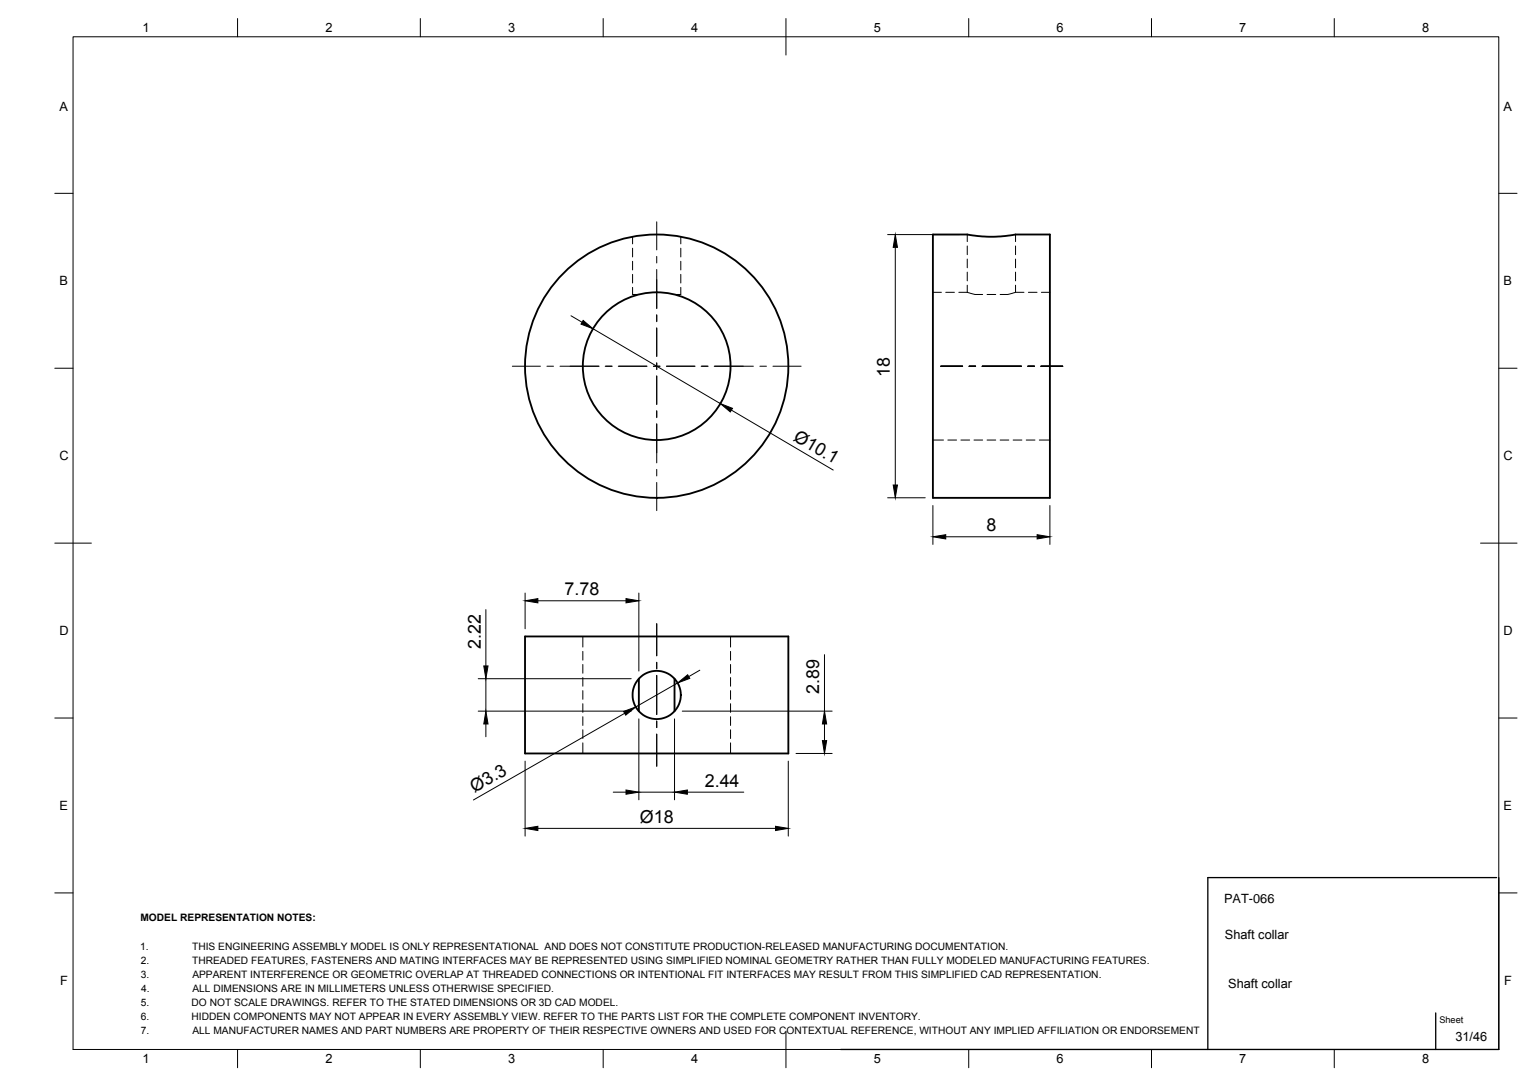
ISO-10303-21;
HEADER;
/* Generated by software containing ST-Developer
 * from STEP Tools, Inc. (www.steptools.com) 
 */

FILE_DESCRIPTION(
/* description */ ('Lever-operated bar clamp (toggle)'),
/* implementation_level */ '2;1');

FILE_NAME(
/* name */ 'Shaft collar.step',
/* time_stamp */ '2026-10-28T03:25:02-07:00',
/* author */ (''),
/* organization */ (''),
/* preprocessor_version */ 'ST-DEVELOPER v20.2',
/* originating_system */ 'Autodesk Translation Framework v15.17.0.0',
/* authorisation */ '');

FILE_SCHEMA (('AUTOMOTIVE_DESIGN { 1 0 10303 214 3 1 1 }'));
ENDSEC;

DATA;
#10=MECHANICAL_DESIGN_GEOMETRIC_PRESENTATION_REPRESENTATION('',(#440),#12413);
#281=B_SPLINE_CURVE_WITH_KNOTS('',3,(#11610,#11611,#11612,#11613,#11614,
#11615,#11616,#11617,#11618,#11619,#11620,#11621,#11622,#11623),
 .UNSPECIFIED.,.F.,.F.,(4,2,2,2,2,2,4),(0.618551524396288,0.626563103102763,
0.689203386094986,0.751843669087208,0.814483952079431,0.877124235071654,
0.88513581377813),.UNSPECIFIED.);
#282=B_SPLINE_CURVE_WITH_KNOTS('',3,(#11629,#11630,#11631,#11632,#11633,
#11634,#11635,#11636,#11637,#11638,#11639,#11640,#11641,#11642,#11643,#11644,
#11645,#11646),.UNSPECIFIED.,.F.,.F.,(4,2,2,2,2,2,2,2,4),(0.,0.0623062782223138,
0.124612556444628,0.186916384615148,0.249220212785668,0.311524040956189,
0.373827869126709,0.436134147349023,0.498440425571337),.UNSPECIFIED.);
#283=B_SPLINE_CURVE_WITH_KNOTS('',3,(#11647,#11648,#11649,#11650,#11651,
#11652,#11653,#11654,#11655,#11656,#11657,#11658,#11659,#11660,#11661,#11662,
#11663,#11664),.UNSPECIFIED.,.F.,.F.,(4,2,2,2,2,2,2,2,4),(0.498440425571337,
0.560746703793651,0.623052982015964,0.685356810186485,0.747660638357005,
0.809964466527525,0.872268294698046,0.93457457292036,0.996880851142673),
 .UNSPECIFIED.);
#284=B_SPLINE_CURVE_WITH_KNOTS('',3,(#11667,#11668,#11669,#11670,#11671,
#11672,#11673,#11674,#11675,#11676,#11677,#11678,#11679,#11680),
 .UNSPECIFIED.,.F.,.F.,(4,2,2,2,2,2,4),(0.117322411671483,0.125333990377957,
0.18797427337018,0.250614556362403,0.313254839354626,0.375895122346849,
0.383906701053325),.UNSPECIFIED.);
#356=SHAPE_REPRESENTATION_RELATIONSHIP('SRR','None',#12598,#394);
#394=ADVANCED_BREP_SHAPE_REPRESENTATION('',(#485),#12395);
#440=STYLED_ITEM('',(#12869),#485);
#485=MANIFOLD_SOLID_BREP('Body1',#6601);
#617=FACE_BOUND('',#1683,.T.);
#618=FACE_BOUND('',#1685,.T.);
#619=FACE_BOUND('',#1687,.T.);
#620=FACE_BOUND('',#1689,.T.);
#798=PLANE('',#7591);
#799=PLANE('',#7596);
#800=PLANE('',#7603);
#801=PLANE('',#7604);
#1156=FACE_OUTER_BOUND('',#1679,.T.);
#1157=FACE_OUTER_BOUND('',#1680,.T.);
#1158=FACE_OUTER_BOUND('',#1681,.T.);
#1159=FACE_OUTER_BOUND('',#1682,.T.);
#1160=FACE_OUTER_BOUND('',#1684,.T.);
#1161=FACE_OUTER_BOUND('',#1686,.T.);
#1162=FACE_OUTER_BOUND('',#1688,.T.);
#1679=EDGE_LOOP('',(#5513,#5514));
#1680=EDGE_LOOP('',(#5515,#5516,#5517,#5518,#5519,#5520,#5521,#5522,#5523));
#1681=EDGE_LOOP('',(#5524,#5525,#5526));
#1682=EDGE_LOOP('',(#5527,#5528,#5529,#5530));
#1683=EDGE_LOOP('',(#5531,#5532,#5533,#5534));
#1684=EDGE_LOOP('',(#5535,#5536,#5537,#5538));
#1685=EDGE_LOOP('',(#5539,#5540));
#1686=EDGE_LOOP('',(#5541));
#1687=EDGE_LOOP('',(#5542));
#1688=EDGE_LOOP('',(#5543));
#1689=EDGE_LOOP('',(#5544));
#2130=LINE('',#11606,#2571);
#2131=LINE('',#11627,#2572);
#2132=LINE('',#11682,#2573);
#2133=LINE('',#11687,#2574);
#2134=LINE('',#11693,#2575);
#2571=VECTOR('',#9279,1.);
#2572=VECTOR('',#9286,0.164999999999999);
#2573=VECTOR('',#9291,1.);
#2574=VECTOR('',#9296,0.505);
#2575=VECTOR('',#9303,0.9);
#2982=CIRCLE('',#7592,0.164999999999999);
#2983=CIRCLE('',#7594,0.164999999999999);
#2984=CIRCLE('',#7595,0.164999999999999);
#2985=CIRCLE('',#7598,0.505);
#2986=CIRCLE('',#7599,0.505);
#2987=CIRCLE('',#7601,0.9);
#2988=CIRCLE('',#7602,0.9);
#3445=VERTEX_POINT('',#11604);
#3446=VERTEX_POINT('',#11605);
#3447=VERTEX_POINT('',#11609);
#3448=VERTEX_POINT('',#11624);
#3449=VERTEX_POINT('',#11626);
#3450=VERTEX_POINT('',#11628);
#3451=VERTEX_POINT('',#11665);
#3452=VERTEX_POINT('',#11684);
#3453=VERTEX_POINT('',#11686);
#3454=VERTEX_POINT('',#11690);
#3455=VERTEX_POINT('',#11692);
#4161=EDGE_CURVE('',#3445,#3446,#2130,.T.);
#4162=EDGE_CURVE('',#3445,#3446,#2982,.T.);
#4163=EDGE_CURVE('',#3447,#3445,#281,.T.);
#4164=EDGE_CURVE('',#3448,#3447,#2983,.T.);
#4165=EDGE_CURVE('',#3448,#3449,#2131,.T.);
#4166=EDGE_CURVE('',#3450,#3449,#282,.T.);
#4167=EDGE_CURVE('',#3449,#3450,#283,.T.);
#4168=EDGE_CURVE('',#3451,#3448,#2984,.T.);
#4169=EDGE_CURVE('',#3446,#3451,#284,.T.);
#4170=EDGE_CURVE('',#3451,#3447,#2132,.T.);
#4171=EDGE_CURVE('',#3452,#3452,#2985,.T.);
#4172=EDGE_CURVE('',#3452,#3453,#2133,.T.);
#4173=EDGE_CURVE('',#3453,#3453,#2986,.T.);
#4174=EDGE_CURVE('',#3454,#3454,#2987,.T.);
#4175=EDGE_CURVE('',#3454,#3455,#2134,.T.);
#4176=EDGE_CURVE('',#3455,#3455,#2988,.T.);
#5513=ORIENTED_EDGE('',*,*,#4161,.F.);
#5514=ORIENTED_EDGE('',*,*,#4162,.T.);
#5515=ORIENTED_EDGE('',*,*,#4163,.F.);
#5516=ORIENTED_EDGE('',*,*,#4164,.F.);
#5517=ORIENTED_EDGE('',*,*,#4165,.T.);
#5518=ORIENTED_EDGE('',*,*,#4166,.F.);
#5519=ORIENTED_EDGE('',*,*,#4167,.F.);
#5520=ORIENTED_EDGE('',*,*,#4165,.F.);
#5521=ORIENTED_EDGE('',*,*,#4168,.F.);
#5522=ORIENTED_EDGE('',*,*,#4169,.F.);
#5523=ORIENTED_EDGE('',*,*,#4162,.F.);
#5524=ORIENTED_EDGE('',*,*,#4170,.F.);
#5525=ORIENTED_EDGE('',*,*,#4168,.T.);
#5526=ORIENTED_EDGE('',*,*,#4164,.T.);
#5527=ORIENTED_EDGE('',*,*,#4171,.F.);
#5528=ORIENTED_EDGE('',*,*,#4172,.T.);
#5529=ORIENTED_EDGE('',*,*,#4173,.T.);
#5530=ORIENTED_EDGE('',*,*,#4172,.F.);
#5531=ORIENTED_EDGE('',*,*,#4169,.T.);
#5532=ORIENTED_EDGE('',*,*,#4170,.T.);
#5533=ORIENTED_EDGE('',*,*,#4163,.T.);
#5534=ORIENTED_EDGE('',*,*,#4161,.T.);
#5535=ORIENTED_EDGE('',*,*,#4174,.F.);
#5536=ORIENTED_EDGE('',*,*,#4175,.T.);
#5537=ORIENTED_EDGE('',*,*,#4176,.T.);
#5538=ORIENTED_EDGE('',*,*,#4175,.F.);
#5539=ORIENTED_EDGE('',*,*,#4166,.T.);
#5540=ORIENTED_EDGE('',*,*,#4167,.T.);
#5541=ORIENTED_EDGE('',*,*,#4174,.T.);
#5542=ORIENTED_EDGE('',*,*,#4171,.T.);
#5543=ORIENTED_EDGE('',*,*,#4176,.F.);
#5544=ORIENTED_EDGE('',*,*,#4173,.F.);
#6125=CYLINDRICAL_SURFACE('',#7593,0.164999999999999);
#6126=CYLINDRICAL_SURFACE('',#7597,0.505);
#6127=CYLINDRICAL_SURFACE('',#7600,0.9);
#6431=ADVANCED_FACE('',(#1156),#798,.T.);
#6432=ADVANCED_FACE('',(#1157),#6125,.F.);
#6433=ADVANCED_FACE('',(#1158),#799,.T.);
#6434=ADVANCED_FACE('',(#1159,#617),#6126,.F.);
#6435=ADVANCED_FACE('',(#1160,#618),#6127,.T.);
#6436=ADVANCED_FACE('',(#1161,#619),#800,.T.);
#6437=ADVANCED_FACE('',(#1162,#620),#801,.F.);
#6601=CLOSED_SHELL('',(#6431,#6432,#6433,#6434,#6435,#6436,#6437));
#7590=AXIS2_PLACEMENT_3D('',#11602,#9275,#9276);
#7591=AXIS2_PLACEMENT_3D('',#11603,#9277,#9278);
#7592=AXIS2_PLACEMENT_3D('',#11607,#9280,#9281);
#7593=AXIS2_PLACEMENT_3D('',#11608,#9282,#9283);
#7594=AXIS2_PLACEMENT_3D('',#11625,#9284,#9285);
#7595=AXIS2_PLACEMENT_3D('',#11666,#9287,#9288);
#7596=AXIS2_PLACEMENT_3D('',#11681,#9289,#9290);
#7597=AXIS2_PLACEMENT_3D('',#11683,#9292,#9293);
#7598=AXIS2_PLACEMENT_3D('',#11685,#9294,#9295);
#7599=AXIS2_PLACEMENT_3D('',#11688,#9297,#9298);
#7600=AXIS2_PLACEMENT_3D('',#11689,#9299,#9300);
#7601=AXIS2_PLACEMENT_3D('',#11691,#9301,#9302);
#7602=AXIS2_PLACEMENT_3D('',#11694,#9304,#9305);
#7603=AXIS2_PLACEMENT_3D('',#11695,#9306,#9307);
#7604=AXIS2_PLACEMENT_3D('',#11696,#9308,#9309);
#9275=DIRECTION('axis',(0.,0.,1.));
#9276=DIRECTION('refdir',(1.,0.,0.));
#9277=DIRECTION('center_axis',(1.,0.,0.));
#9278=DIRECTION('ref_axis',(0.,0.,-1.));
#9279=DIRECTION('',(0.,1.,0.));
#9280=DIRECTION('center_axis',(1.,0.,0.));
#9281=DIRECTION('ref_axis',(0.,0.,-1.));
#9282=DIRECTION('center_axis',(1.,0.,0.));
#9283=DIRECTION('ref_axis',(0.,0.,-1.));
#9284=DIRECTION('center_axis',(1.,0.,0.));
#9285=DIRECTION('ref_axis',(0.,0.,-1.));
#9286=DIRECTION('',(1.,0.,0.));
#9287=DIRECTION('center_axis',(1.,0.,0.));
#9288=DIRECTION('ref_axis',(0.,0.,-1.));
#9289=DIRECTION('center_axis',(1.,0.,0.));
#9290=DIRECTION('ref_axis',(0.,0.,-1.));
#9291=DIRECTION('',(0.,-1.,0.));
#9292=DIRECTION('center_axis',(0.,1.,0.));
#9293=DIRECTION('ref_axis',(1.,0.,0.));
#9294=DIRECTION('center_axis',(0.,-1.,0.));
#9295=DIRECTION('ref_axis',(1.,0.,0.));
#9296=DIRECTION('',(0.,-1.,0.));
#9297=DIRECTION('center_axis',(0.,-1.,0.));
#9298=DIRECTION('ref_axis',(1.,0.,0.));
#9299=DIRECTION('center_axis',(0.,1.,0.));
#9300=DIRECTION('ref_axis',(1.,0.,0.));
#9301=DIRECTION('center_axis',(0.,1.,0.));
#9302=DIRECTION('ref_axis',(1.,0.,0.));
#9303=DIRECTION('',(0.,-1.,0.));
#9304=DIRECTION('center_axis',(0.,1.,0.));
#9305=DIRECTION('ref_axis',(1.,0.,0.));
#9306=DIRECTION('center_axis',(0.,1.,0.));
#9307=DIRECTION('ref_axis',(1.,0.,0.));
#9308=DIRECTION('center_axis',(0.,1.,0.));
#9309=DIRECTION('ref_axis',(1.,0.,0.));
#11602=CARTESIAN_POINT('',(0.,0.,0.));
#11603=CARTESIAN_POINT('Origin',(-3.51,1.4,11.));
#11604=CARTESIAN_POINT('',(-3.51,1.28909463493591,10.8778320827713));
#11605=CARTESIAN_POINT('',(-3.51,1.51090536506409,10.8778320827713));
#11606=CARTESIAN_POINT('',(-3.51,1.,10.8778320827713));
#11607=CARTESIAN_POINT('Origin',(-3.51,1.4,11.));
#11608=CARTESIAN_POINT('Origin',(-3.51,1.4,11.));
#11609=CARTESIAN_POINT('',(-3.51,1.28909463493591,11.1221679172287));
#11610=CARTESIAN_POINT('Ctrl Pts',(-3.51,1.28909463493591,11.1221679172287));
#11611=CARTESIAN_POINT('Ctrl Pts',(-3.50955146832001,1.28711294069536,11.1203689136263));
#11612=CARTESIAN_POINT('Ctrl Pts',(-3.50910475462832,1.28518965877367,11.1185348965652));
#11613=CARTESIAN_POINT('Ctrl Pts',(-3.50520498446835,1.2687667552278,11.1021119930194));
#11614=CARTESIAN_POINT('Ctrl Pts',(-3.50155748539241,1.25609154388858,11.0836597150224));
#11615=CARTESIAN_POINT('Ctrl Pts',(-3.49642218023894,1.23920409039234,11.0430495960472));
#11616=CARTESIAN_POINT('Ctrl Pts',(-3.495,1.235,11.0208800943307));
#11617=CARTESIAN_POINT('Ctrl Pts',(-3.495,1.235,10.9791199056693));
#11618=CARTESIAN_POINT('Ctrl Pts',(-3.49642218023894,1.23920409039234,10.9569504039528));
#11619=CARTESIAN_POINT('Ctrl Pts',(-3.50155748539241,1.25609154388858,10.9163402849776));
#11620=CARTESIAN_POINT('Ctrl Pts',(-3.50520498446835,1.2687667552278,10.8978880069806));
#11621=CARTESIAN_POINT('Ctrl Pts',(-3.50910475462832,1.28518965877367,10.8814651034348));
#11622=CARTESIAN_POINT('Ctrl Pts',(-3.50955146832001,1.28711294069536,10.8796310863737));
#11623=CARTESIAN_POINT('Ctrl Pts',(-3.51,1.28909463493591,10.8778320827713));
#11624=CARTESIAN_POINT('',(-3.51,1.4,11.165));
#11625=CARTESIAN_POINT('Origin',(-3.51,1.4,11.));
#11626=CARTESIAN_POINT('',(-3.11525427381648,1.4,11.165));
#11627=CARTESIAN_POINT('',(-3.51,1.4,11.165));
#11628=CARTESIAN_POINT('',(-3.11525427381648,1.4,10.835));
#11629=CARTESIAN_POINT('Ctrl Pts',(-3.11525427381648,1.4,10.835));
#11630=CARTESIAN_POINT('Ctrl Pts',(-3.11525427381648,1.37923124059256,10.835));
#11631=CARTESIAN_POINT('Ctrl Pts',(-3.11444724049474,1.35711110492666,10.8391602809924));
#11632=CARTESIAN_POINT('Ctrl Pts',(-3.11155135184996,1.31647293736623,10.8560135297833));
#11633=CARTESIAN_POINT('Ctrl Pts',(-3.10950639514836,1.29795075602263,10.8687040061858));
#11634=CARTESIAN_POINT('Ctrl Pts',(-3.10568276567606,1.26870458121656,10.8979501809919));
#11635=CARTESIAN_POINT('Ctrl Pts',(-3.10365291110046,1.25601365401642,10.9164726079093));
#11636=CARTESIAN_POINT('Ctrl Pts',(-3.10079172813942,1.23916007816136,10.9571116239066));
#11637=CARTESIAN_POINT('Ctrl Pts',(-3.1,1.235,10.9792320572765));
#11638=CARTESIAN_POINT('Ctrl Pts',(-3.1,1.235,11.0207679427235));
#11639=CARTESIAN_POINT('Ctrl Pts',(-3.10079172813942,1.23916007816136,11.0428883760934));
#11640=CARTESIAN_POINT('Ctrl Pts',(-3.10365291110046,1.25601365401642,11.0835273920907));
#11641=CARTESIAN_POINT('Ctrl Pts',(-3.10568276567606,1.26870458121656,11.1020498190081));
#11642=CARTESIAN_POINT('Ctrl Pts',(-3.10950639514836,1.29795075602263,11.1312959938142));
#11643=CARTESIAN_POINT('Ctrl Pts',(-3.11155135184996,1.31647293736623,11.1439864702167));
#11644=CARTESIAN_POINT('Ctrl Pts',(-3.11444724049474,1.35711110492666,11.1608397190076));
#11645=CARTESIAN_POINT('Ctrl Pts',(-3.11525427381648,1.37923124059256,11.165));
#11646=CARTESIAN_POINT('Ctrl Pts',(-3.11525427381648,1.4,11.165));
#11647=CARTESIAN_POINT('Ctrl Pts',(-3.11525427381648,1.4,11.165));
#11648=CARTESIAN_POINT('Ctrl Pts',(-3.11525427381648,1.42076875940744,11.165));
#11649=CARTESIAN_POINT('Ctrl Pts',(-3.11444724049474,1.44288889507334,11.1608397190076));
#11650=CARTESIAN_POINT('Ctrl Pts',(-3.11155135184996,1.48352706263377,11.1439864702167));
#11651=CARTESIAN_POINT('Ctrl Pts',(-3.10950639514836,1.50204924397737,11.1312959938142));
#11652=CARTESIAN_POINT('Ctrl Pts',(-3.10568276567606,1.53129541878343,11.1020498190081));
#11653=CARTESIAN_POINT('Ctrl Pts',(-3.10365291110046,1.54398634598358,11.0835273920907));
#11654=CARTESIAN_POINT('Ctrl Pts',(-3.10079172813942,1.56083992183864,11.0428883760934));
#11655=CARTESIAN_POINT('Ctrl Pts',(-3.1,1.565,11.0207679427235));
#11656=CARTESIAN_POINT('Ctrl Pts',(-3.1,1.565,10.9792320572765));
#11657=CARTESIAN_POINT('Ctrl Pts',(-3.10079172813942,1.56083992183864,10.9571116239066));
#11658=CARTESIAN_POINT('Ctrl Pts',(-3.10365291110046,1.54398634598358,10.9164726079093));
#11659=CARTESIAN_POINT('Ctrl Pts',(-3.10568276567606,1.53129541878343,10.8979501809919));
#11660=CARTESIAN_POINT('Ctrl Pts',(-3.10950639514836,1.50204924397737,10.8687040061858));
#11661=CARTESIAN_POINT('Ctrl Pts',(-3.11155135184996,1.48352706263377,10.8560135297833));
#11662=CARTESIAN_POINT('Ctrl Pts',(-3.11444724049474,1.44288889507334,10.8391602809924));
#11663=CARTESIAN_POINT('Ctrl Pts',(-3.11525427381648,1.42076875940744,10.835));
#11664=CARTESIAN_POINT('Ctrl Pts',(-3.11525427381648,1.4,10.835));
#11665=CARTESIAN_POINT('',(-3.51,1.51090536506409,11.1221679172287));
#11666=CARTESIAN_POINT('Origin',(-3.51,1.4,11.));
#11667=CARTESIAN_POINT('Ctrl Pts',(-3.51,1.51090536506409,10.8778320827713));
#11668=CARTESIAN_POINT('Ctrl Pts',(-3.50955146832001,1.51288705930464,10.8796310863737));
#11669=CARTESIAN_POINT('Ctrl Pts',(-3.50910475462832,1.51481034122633,10.8814651034348));
#11670=CARTESIAN_POINT('Ctrl Pts',(-3.50520498446835,1.5312332447722,10.8978880069806));
#11671=CARTESIAN_POINT('Ctrl Pts',(-3.50155748539241,1.54390845611142,10.9163402849776));
#11672=CARTESIAN_POINT('Ctrl Pts',(-3.49642218023894,1.56079590960766,10.9569504039528));
#11673=CARTESIAN_POINT('Ctrl Pts',(-3.495,1.565,10.9791199056693));
#11674=CARTESIAN_POINT('Ctrl Pts',(-3.495,1.565,11.0208800943307));
#11675=CARTESIAN_POINT('Ctrl Pts',(-3.49642218023894,1.56079590960766,11.0430495960472));
#11676=CARTESIAN_POINT('Ctrl Pts',(-3.50155748539241,1.54390845611142,11.0836597150224));
#11677=CARTESIAN_POINT('Ctrl Pts',(-3.50520498446835,1.5312332447722,11.1021119930194));
#11678=CARTESIAN_POINT('Ctrl Pts',(-3.50910475462832,1.51481034122633,11.1185348965652));
#11679=CARTESIAN_POINT('Ctrl Pts',(-3.50955146832001,1.51288705930464,11.1203689136263));
#11680=CARTESIAN_POINT('Ctrl Pts',(-3.51,1.51090536506409,11.1221679172287));
#11681=CARTESIAN_POINT('Origin',(-3.51,1.4,11.));
#11682=CARTESIAN_POINT('',(-3.51,1.,11.1221679172287));
#11683=CARTESIAN_POINT('Origin',(-4.,1.,11.));
#11684=CARTESIAN_POINT('',(-4.505,1.8,11.));
#11685=CARTESIAN_POINT('Origin',(-4.,1.8,11.));
#11686=CARTESIAN_POINT('',(-4.505,1.,11.));
#11687=CARTESIAN_POINT('',(-4.505,1.,11.));
#11688=CARTESIAN_POINT('Origin',(-4.,1.,11.));
#11689=CARTESIAN_POINT('Origin',(-4.,1.,11.));
#11690=CARTESIAN_POINT('',(-4.9,1.8,11.));
#11691=CARTESIAN_POINT('Origin',(-4.,1.8,11.));
#11692=CARTESIAN_POINT('',(-4.9,1.,11.));
#11693=CARTESIAN_POINT('',(-4.9,1.,11.));
#11694=CARTESIAN_POINT('Origin',(-4.,1.,11.));
#11695=CARTESIAN_POINT('Origin',(-4.,1.8,11.));
#11696=CARTESIAN_POINT('Origin',(-4.,1.,11.));
#12349=UNCERTAINTY_MEASURE_WITH_UNIT(LENGTH_MEASURE(0.001),#12414,
'DISTANCE_ACCURACY_VALUE',
'Maximum model space distance between geometric entities at asserted c
onnectivities');
#12367=UNCERTAINTY_MEASURE_WITH_UNIT(LENGTH_MEASURE(0.001),#12414,
'DISTANCE_ACCURACY_VALUE',
'Maximum model space distance between geometric entities at asserted c
onnectivities');
#12395=(
GEOMETRIC_REPRESENTATION_CONTEXT(3)
GLOBAL_UNCERTAINTY_ASSIGNED_CONTEXT((#12349))
GLOBAL_UNIT_ASSIGNED_CONTEXT((#12414,#12416,#12417))
REPRESENTATION_CONTEXT('','3D')
);
#12413=(
GEOMETRIC_REPRESENTATION_CONTEXT(3)
GLOBAL_UNCERTAINTY_ASSIGNED_CONTEXT((#12367))
GLOBAL_UNIT_ASSIGNED_CONTEXT((#12414,#12416,#12417))
REPRESENTATION_CONTEXT('','3D')
);
#12414=(
LENGTH_UNIT()
NAMED_UNIT(*)
SI_UNIT(.CENTI.,.METRE.)
);
#12416=(
NAMED_UNIT(*)
PLANE_ANGLE_UNIT()
SI_UNIT($,.RADIAN.)
);
#12417=(
NAMED_UNIT(*)
SI_UNIT($,.STERADIAN.)
SOLID_ANGLE_UNIT()
);
#12445=SHAPE_DEFINITION_REPRESENTATION(#12497,#12598);
#12497=PRODUCT_DEFINITION_SHAPE('',$,#12644);
#12598=SHAPE_REPRESENTATION('',(#7590),#12395);
#12616=PRODUCT_DEFINITION_CONTEXT('part definition',#12753,'design');
#12644=PRODUCT_DEFINITION('Shaft collar','Shaft collar',#12689,#12616);
#12689=PRODUCT_DEFINITION_FORMATION('',$,#12782);
#12753=APPLICATION_CONTEXT(
'Core Data for Automotive Mechanical Design Process');
#12754=PRODUCT_CONTEXT('part definition',#12753,'mechanical');
#12782=PRODUCT('Shaft collar','Shaft collar','Shaft collar',(#12754));
#12863=COLOUR_RGB('Grey',0.48,0.52,0.57);
#12864=FILL_AREA_STYLE_COLOUR('',#12863);
#12865=FILL_AREA_STYLE('',(#12864));
#12866=SURFACE_STYLE_FILL_AREA(#12865);
#12867=SURFACE_SIDE_STYLE('',(#12866));
#12868=SURFACE_STYLE_USAGE(.BOTH.,#12867);
#12869=PRESENTATION_STYLE_ASSIGNMENT((#12868));
ENDSEC;
END-ISO-10303-21;
